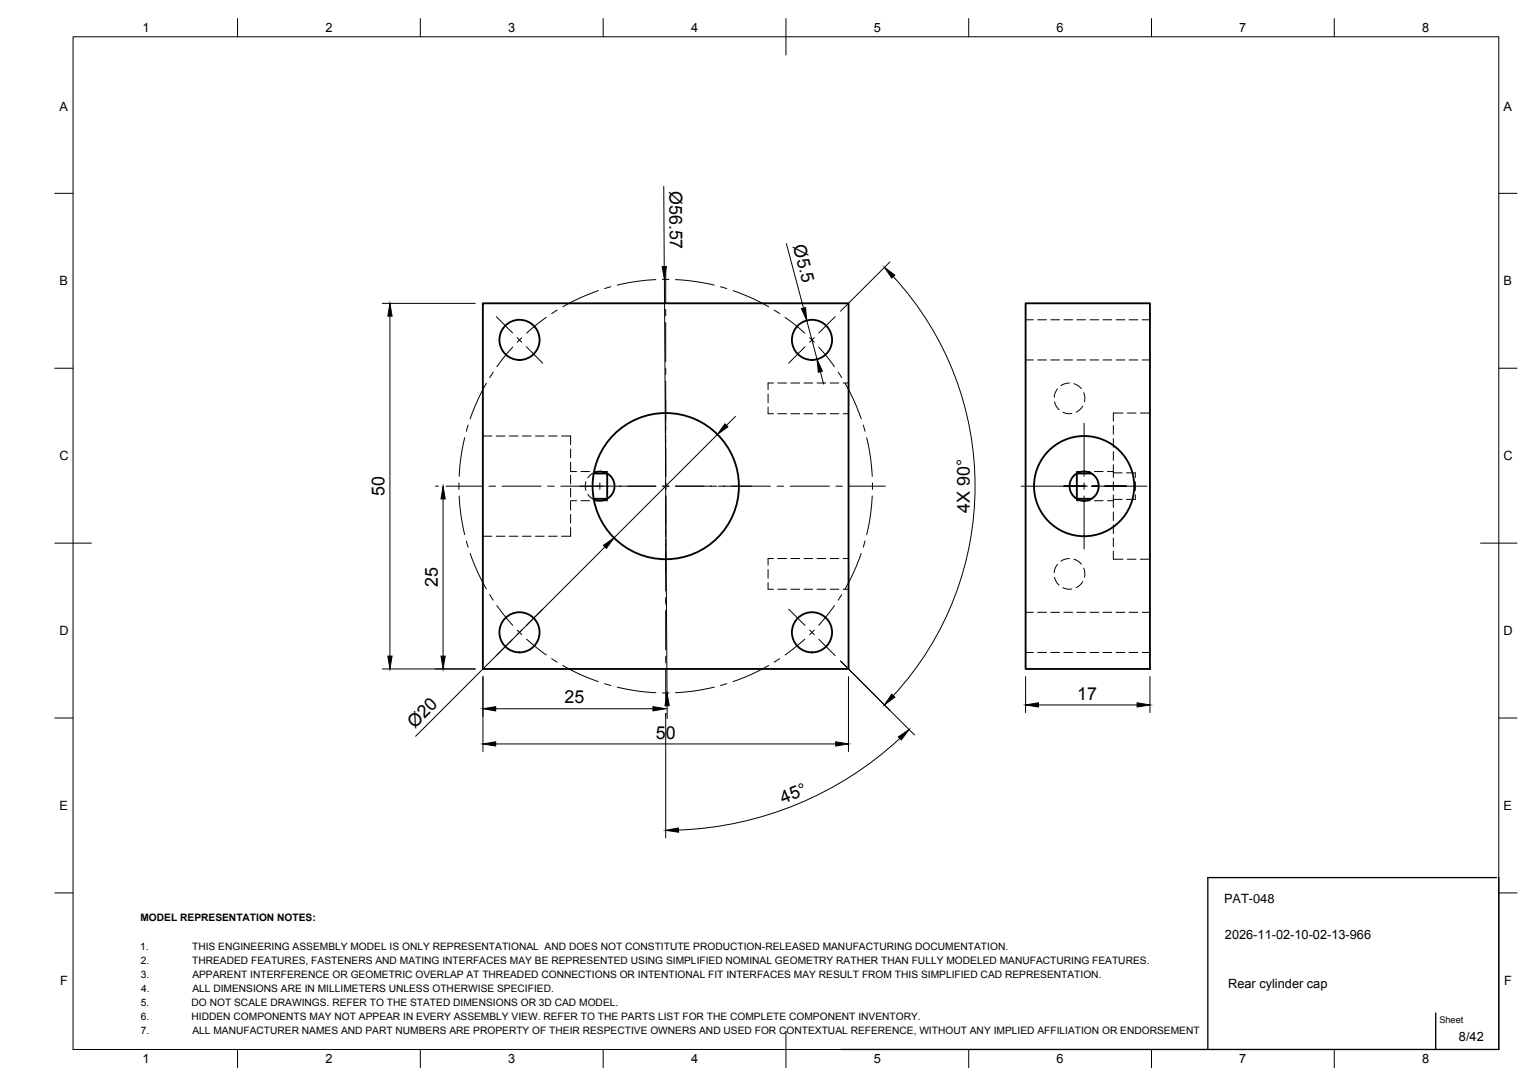
ISO-10303-21;
HEADER;
/* Generated by software containing ST-Developer
 * from STEP Tools, Inc. (www.steptools.com) 
 */

FILE_DESCRIPTION(
/* description */ ('Guided pneumatic stop gate'),
/* implementation_level */ '2;1');

FILE_NAME(
/* name */ 'Rear cylinder cap.step',
/* time_stamp */ '2026-10-27T21:43:45-07:00',
/* author */ (''),
/* organization */ (''),
/* preprocessor_version */ 'ST-DEVELOPER v20.2',
/* originating_system */ 'Autodesk Translation Framework v15.17.0.0',
/* authorisation */ '');

FILE_SCHEMA (('AUTOMOTIVE_DESIGN { 1 0 10303 214 3 1 1 }'));
ENDSEC;

DATA;
#10=MECHANICAL_DESIGN_GEOMETRIC_PRESENTATION_REPRESENTATION('',(#538),#14392);
#454=SHAPE_REPRESENTATION_RELATIONSHIP('SRR','None',#14588,#496);
#496=ADVANCED_BREP_SHAPE_REPRESENTATION('',(#580),#14350);
#538=STYLED_ITEM('',(#14877),#580);
#580=MANIFOLD_SOLID_BREP('Body1',#7878);
#640=FACE_BOUND('',#1705,.T.);
#641=FACE_BOUND('',#1712,.T.);
#642=FACE_BOUND('',#1713,.T.);
#643=FACE_BOUND('',#1714,.T.);
#644=FACE_BOUND('',#1715,.T.);
#645=FACE_BOUND('',#1718,.T.);
#646=FACE_BOUND('',#1719,.T.);
#647=FACE_BOUND('',#1720,.T.);
#648=FACE_BOUND('',#1721,.T.);
#649=FACE_BOUND('',#1722,.T.);
#650=FACE_BOUND('',#1725,.T.);
#651=FACE_BOUND('',#1727,.T.);
#652=FACE_BOUND('',#1728,.T.);
#832=ELLIPSE('',#8530,0.282842712474618,0.2);
#833=ELLIPSE('',#8531,0.282842712474618,0.2);
#834=ELLIPSE('',#8532,0.282842712474618,0.2);
#835=ELLIPSE('',#8535,0.282842712474618,0.2);
#836=ELLIPSE('',#8536,0.282842712474618,0.2);
#837=ELLIPSE('',#8538,0.282842712474618,0.2);
#838=ELLIPSE('',#8539,0.282842712474618,0.2);
#880=PLANE('',#8516);
#881=PLANE('',#8520);
#882=PLANE('',#8521);
#883=PLANE('',#8523);
#884=PLANE('',#8525);
#885=PLANE('',#8540);
#886=PLANE('',#8542);
#887=PLANE('',#8544);
#888=PLANE('',#8546);
#889=PLANE('',#8552);
#890=PLANE('',#8558);
#891=PLANE('',#8573);
#892=PLANE('',#8574);
#893=PLANE('',#8575);
#894=PLANE('',#8576);
#895=PLANE('',#8577);
#896=PLANE('',#8578);
#1185=FACE_OUTER_BOUND('',#1685,.T.);
#1186=FACE_OUTER_BOUND('',#1686,.T.);
#1187=FACE_OUTER_BOUND('',#1687,.T.);
#1188=FACE_OUTER_BOUND('',#1688,.T.);
#1189=FACE_OUTER_BOUND('',#1689,.T.);
#1190=FACE_OUTER_BOUND('',#1690,.T.);
#1191=FACE_OUTER_BOUND('',#1691,.T.);
#1192=FACE_OUTER_BOUND('',#1692,.T.);
#1193=FACE_OUTER_BOUND('',#1693,.T.);
#1194=FACE_OUTER_BOUND('',#1694,.T.);
#1195=FACE_OUTER_BOUND('',#1695,.T.);
#1196=FACE_OUTER_BOUND('',#1696,.T.);
#1197=FACE_OUTER_BOUND('',#1697,.T.);
#1198=FACE_OUTER_BOUND('',#1698,.T.);
#1199=FACE_OUTER_BOUND('',#1699,.T.);
#1200=FACE_OUTER_BOUND('',#1700,.T.);
#1201=FACE_OUTER_BOUND('',#1701,.T.);
#1202=FACE_OUTER_BOUND('',#1702,.T.);
#1203=FACE_OUTER_BOUND('',#1703,.T.);
#1204=FACE_OUTER_BOUND('',#1704,.T.);
#1205=FACE_OUTER_BOUND('',#1706,.T.);
#1206=FACE_OUTER_BOUND('',#1707,.T.);
#1207=FACE_OUTER_BOUND('',#1708,.T.);
#1208=FACE_OUTER_BOUND('',#1709,.T.);
#1209=FACE_OUTER_BOUND('',#1710,.T.);
#1210=FACE_OUTER_BOUND('',#1711,.T.);
#1211=FACE_OUTER_BOUND('',#1716,.T.);
#1212=FACE_OUTER_BOUND('',#1717,.T.);
#1213=FACE_OUTER_BOUND('',#1723,.T.);
#1214=FACE_OUTER_BOUND('',#1724,.T.);
#1215=FACE_OUTER_BOUND('',#1726,.T.);
#1685=EDGE_LOOP('',(#5592,#5593,#5594,#5595));
#1686=EDGE_LOOP('',(#5596));
#1687=EDGE_LOOP('',(#5597,#5598,#5599,#5600));
#1688=EDGE_LOOP('',(#5601));
#1689=EDGE_LOOP('',(#5602,#5603));
#1690=EDGE_LOOP('',(#5604,#5605));
#1691=EDGE_LOOP('',(#5606,#5607));
#1692=EDGE_LOOP('',(#5608,#5609,#5610,#5611,#5612,#5613,#5614,#5615,#5616,
#5617,#5618,#5619,#5620));
#1693=EDGE_LOOP('',(#5621,#5622,#5623));
#1694=EDGE_LOOP('',(#5624,#5625,#5626));
#1695=EDGE_LOOP('',(#5627,#5628));
#1696=EDGE_LOOP('',(#5629,#5630));
#1697=EDGE_LOOP('',(#5631,#5632));
#1698=EDGE_LOOP('',(#5633,#5634));
#1699=EDGE_LOOP('',(#5635,#5636,#5637));
#1700=EDGE_LOOP('',(#5638,#5639,#5640));
#1701=EDGE_LOOP('',(#5641,#5642,#5643,#5644,#5645,#5646,#5647,#5648,#5649));
#1702=EDGE_LOOP('',(#5650,#5651,#5652,#5653));
#1703=EDGE_LOOP('',(#5654,#5655,#5656,#5657));
#1704=EDGE_LOOP('',(#5658));
#1705=EDGE_LOOP('',(#5659));
#1706=EDGE_LOOP('',(#5660,#5661,#5662,#5663));
#1707=EDGE_LOOP('',(#5664,#5665,#5666,#5667));
#1708=EDGE_LOOP('',(#5668,#5669,#5670,#5671));
#1709=EDGE_LOOP('',(#5672,#5673,#5674,#5675));
#1710=EDGE_LOOP('',(#5676,#5677,#5678,#5679,#5680,#5681,#5682,#5683));
#1711=EDGE_LOOP('',(#5684,#5685,#5686,#5687));
#1712=EDGE_LOOP('',(#5688));
#1713=EDGE_LOOP('',(#5689));
#1714=EDGE_LOOP('',(#5690));
#1715=EDGE_LOOP('',(#5691));
#1716=EDGE_LOOP('',(#5692,#5693,#5694,#5695));
#1717=EDGE_LOOP('',(#5696,#5697,#5698,#5699));
#1718=EDGE_LOOP('',(#5700));
#1719=EDGE_LOOP('',(#5701));
#1720=EDGE_LOOP('',(#5702));
#1721=EDGE_LOOP('',(#5703));
#1722=EDGE_LOOP('',(#5704));
#1723=EDGE_LOOP('',(#5705,#5706,#5707,#5708));
#1724=EDGE_LOOP('',(#5709,#5710,#5711,#5712));
#1725=EDGE_LOOP('',(#5713));
#1726=EDGE_LOOP('',(#5714,#5715,#5716,#5717));
#1727=EDGE_LOOP('',(#5718));
#1728=EDGE_LOOP('',(#5719));
#2360=LINE('',#12221,#2905);
#2361=LINE('',#12228,#2906);
#2362=LINE('',#12234,#2907);
#2363=LINE('',#12238,#2908);
#2364=LINE('',#12242,#2909);
#2365=LINE('',#12247,#2910);
#2366=LINE('',#12251,#2911);
#2367=LINE('',#12255,#2912);
#2368=LINE('',#12260,#2913);
#2369=LINE('',#12262,#2914);
#2370=LINE('',#12283,#2915);
#2371=LINE('',#12293,#2916);
#2372=LINE('',#12300,#2917);
#2373=LINE('',#12306,#2918);
#2374=LINE('',#12312,#2919);
#2375=LINE('',#12318,#2920);
#2376=LINE('',#12323,#2921);
#2377=LINE('',#12327,#2922);
#2378=LINE('',#12329,#2923);
#2379=LINE('',#12331,#2924);
#2380=LINE('',#12332,#2925);
#2381=LINE('',#12335,#2926);
#2382=LINE('',#12337,#2927);
#2383=LINE('',#12338,#2928);
#2384=LINE('',#12341,#2929);
#2385=LINE('',#12343,#2930);
#2386=LINE('',#12344,#2931);
#2387=LINE('',#12346,#2932);
#2388=LINE('',#12347,#2933);
#2905=VECTOR('',#9725,0.21);
#2906=VECTOR('',#9734,0.21);
#2907=VECTOR('',#9741,1.);
#2908=VECTOR('',#9746,1.);
#2909=VECTOR('',#9751,1.);
#2910=VECTOR('',#9756,1.);
#2911=VECTOR('',#9759,1.);
#2912=VECTOR('',#9762,0.2);
#2913=VECTOR('',#9767,1.);
#2914=VECTOR('',#9768,1.);
#2915=VECTOR('',#9807,0.2);
#2916=VECTOR('',#9820,0.685);
#2917=VECTOR('',#9829,0.275);
#2918=VECTOR('',#9836,0.275);
#2919=VECTOR('',#9843,0.275);
#2920=VECTOR('',#9850,0.275);
#2921=VECTOR('',#9857,1.);
#2922=VECTOR('',#9860,1.);
#2923=VECTOR('',#9861,1.);
#2924=VECTOR('',#9862,1.);
#2925=VECTOR('',#9863,1.);
#2926=VECTOR('',#9866,1.);
#2927=VECTOR('',#9867,1.);
#2928=VECTOR('',#9868,1.);
#2929=VECTOR('',#9871,1.);
#2930=VECTOR('',#9872,1.);
#2931=VECTOR('',#9873,1.);
#2932=VECTOR('',#9876,1.);
#2933=VECTOR('',#9877,1.);
#3417=CIRCLE('',#8514,0.21);
#3418=CIRCLE('',#8515,0.21);
#3419=CIRCLE('',#8518,0.21);
#3420=CIRCLE('',#8519,0.21);
#3421=CIRCLE('',#8522,0.2);
#3422=CIRCLE('',#8524,0.2);
#3423=CIRCLE('',#8526,0.2);
#3424=CIRCLE('',#8528,0.2);
#3425=CIRCLE('',#8529,0.2);
#3426=CIRCLE('',#8533,0.2);
#3427=CIRCLE('',#8541,1.);
#3428=CIRCLE('',#8543,0.2);
#3429=CIRCLE('',#8545,0.2);
#3430=CIRCLE('',#8547,0.2);
#3431=CIRCLE('',#8551,0.2);
#3432=CIRCLE('',#8553,1.);
#3433=CIRCLE('',#8554,1.);
#3434=CIRCLE('',#8556,0.685);
#3435=CIRCLE('',#8557,0.685);
#3436=CIRCLE('',#8560,0.275);
#3437=CIRCLE('',#8561,0.275);
#3438=CIRCLE('',#8563,0.275);
#3439=CIRCLE('',#8564,0.275);
#3440=CIRCLE('',#8566,0.275);
#3441=CIRCLE('',#8567,0.275);
#3442=CIRCLE('',#8569,0.275);
#3443=CIRCLE('',#8570,0.275);
#3444=CIRCLE('',#8572,1.);
#3823=VERTEX_POINT('',#12218);
#3824=VERTEX_POINT('',#12220);
#3825=VERTEX_POINT('',#12225);
#3826=VERTEX_POINT('',#12227);
#3827=VERTEX_POINT('',#12232);
#3828=VERTEX_POINT('',#12233);
#3829=VERTEX_POINT('',#12237);
#3830=VERTEX_POINT('',#12241);
#3831=VERTEX_POINT('',#12245);
#3832=VERTEX_POINT('',#12246);
#3833=VERTEX_POINT('',#12248);
#3834=VERTEX_POINT('',#12250);
#3835=VERTEX_POINT('',#12252);
#3836=VERTEX_POINT('',#12254);
#3837=VERTEX_POINT('',#12256);
#3838=VERTEX_POINT('',#12258);
#3839=VERTEX_POINT('',#12261);
#3840=VERTEX_POINT('',#12282);
#3841=VERTEX_POINT('',#12286);
#3842=VERTEX_POINT('',#12290);
#3843=VERTEX_POINT('',#12292);
#3844=VERTEX_POINT('',#12297);
#3845=VERTEX_POINT('',#12299);
#3846=VERTEX_POINT('',#12303);
#3847=VERTEX_POINT('',#12305);
#3848=VERTEX_POINT('',#12309);
#3849=VERTEX_POINT('',#12311);
#3850=VERTEX_POINT('',#12315);
#3851=VERTEX_POINT('',#12317);
#3852=VERTEX_POINT('',#12321);
#3853=VERTEX_POINT('',#12325);
#3854=VERTEX_POINT('',#12326);
#3855=VERTEX_POINT('',#12328);
#3856=VERTEX_POINT('',#12330);
#3857=VERTEX_POINT('',#12334);
#3858=VERTEX_POINT('',#12336);
#3859=VERTEX_POINT('',#12340);
#3860=VERTEX_POINT('',#12342);
#4494=EDGE_CURVE('',#3823,#3823,#3417,.T.);
#4495=EDGE_CURVE('',#3823,#3824,#2360,.T.);
#4496=EDGE_CURVE('',#3824,#3824,#3418,.T.);
#4497=EDGE_CURVE('',#3825,#3825,#3419,.T.);
#4498=EDGE_CURVE('',#3825,#3826,#2361,.T.);
#4499=EDGE_CURVE('',#3826,#3826,#3420,.T.);
#4500=EDGE_CURVE('',#3827,#3828,#2362,.T.);
#4501=EDGE_CURVE('',#3828,#3827,#3421,.T.);
#4502=EDGE_CURVE('',#3828,#3829,#2363,.T.);
#4503=EDGE_CURVE('',#3829,#3828,#3422,.T.);
#4504=EDGE_CURVE('',#3830,#3827,#2364,.T.);
#4505=EDGE_CURVE('',#3827,#3830,#3423,.T.);
#4506=EDGE_CURVE('',#3831,#3832,#2365,.T.);
#4507=EDGE_CURVE('',#3833,#3831,#3424,.T.);
#4508=EDGE_CURVE('',#3834,#3833,#2366,.T.);
#4509=EDGE_CURVE('',#3835,#3834,#3425,.T.);
#4510=EDGE_CURVE('',#3835,#3836,#2367,.T.);
#4511=EDGE_CURVE('',#3837,#3836,#832,.T.);
#4512=EDGE_CURVE('',#3838,#3837,#833,.T.);
#4513=EDGE_CURVE('',#3828,#3838,#2368,.T.);
#4514=EDGE_CURVE('',#3839,#3827,#2369,.T.);
#4515=EDGE_CURVE('',#3836,#3839,#834,.T.);
#4516=EDGE_CURVE('',#3832,#3835,#3426,.T.);
#4517=EDGE_CURVE('',#3829,#3837,#835,.T.);
#4518=EDGE_CURVE('',#3837,#3828,#836,.T.);
#4519=EDGE_CURVE('',#3836,#3830,#837,.T.);
#4520=EDGE_CURVE('',#3827,#3836,#838,.T.);
#4521=EDGE_CURVE('',#3833,#3831,#3427,.T.);
#4522=EDGE_CURVE('',#3828,#3827,#3428,.T.);
#4523=EDGE_CURVE('',#3838,#3828,#3429,.T.);
#4524=EDGE_CURVE('',#3827,#3839,#3430,.T.);
#4525=EDGE_CURVE('',#3836,#3840,#2370,.T.);
#4526=EDGE_CURVE('',#3840,#3840,#3431,.T.);
#4527=EDGE_CURVE('',#3841,#3834,#3432,.T.);
#4528=EDGE_CURVE('',#3832,#3841,#3433,.T.);
#4529=EDGE_CURVE('',#3842,#3842,#3434,.T.);
#4530=EDGE_CURVE('',#3842,#3843,#2371,.T.);
#4531=EDGE_CURVE('',#3843,#3843,#3435,.T.);
#4532=EDGE_CURVE('',#3844,#3844,#3436,.T.);
#4533=EDGE_CURVE('',#3844,#3845,#2372,.T.);
#4534=EDGE_CURVE('',#3845,#3845,#3437,.T.);
#4535=EDGE_CURVE('',#3846,#3846,#3438,.T.);
#4536=EDGE_CURVE('',#3846,#3847,#2373,.T.);
#4537=EDGE_CURVE('',#3847,#3847,#3439,.T.);
#4538=EDGE_CURVE('',#3848,#3848,#3440,.T.);
#4539=EDGE_CURVE('',#3848,#3849,#2374,.T.);
#4540=EDGE_CURVE('',#3849,#3849,#3441,.T.);
#4541=EDGE_CURVE('',#3850,#3850,#3442,.T.);
#4542=EDGE_CURVE('',#3850,#3851,#2375,.T.);
#4543=EDGE_CURVE('',#3851,#3851,#3443,.T.);
#4544=EDGE_CURVE('',#3852,#3852,#3444,.T.);
#4545=EDGE_CURVE('',#3852,#3841,#2376,.T.);
#4546=EDGE_CURVE('',#3853,#3854,#2377,.T.);
#4547=EDGE_CURVE('',#3854,#3855,#2378,.T.);
#4548=EDGE_CURVE('',#3856,#3855,#2379,.T.);
#4549=EDGE_CURVE('',#3853,#3856,#2380,.T.);
#4550=EDGE_CURVE('',#3857,#3853,#2381,.T.);
#4551=EDGE_CURVE('',#3858,#3856,#2382,.T.);
#4552=EDGE_CURVE('',#3857,#3858,#2383,.T.);
#4553=EDGE_CURVE('',#3859,#3857,#2384,.T.);
#4554=EDGE_CURVE('',#3860,#3858,#2385,.T.);
#4555=EDGE_CURVE('',#3859,#3860,#2386,.T.);
#4556=EDGE_CURVE('',#3854,#3859,#2387,.T.);
#4557=EDGE_CURVE('',#3855,#3860,#2388,.T.);
#5592=ORIENTED_EDGE('',*,*,#4494,.F.);
#5593=ORIENTED_EDGE('',*,*,#4495,.T.);
#5594=ORIENTED_EDGE('',*,*,#4496,.T.);
#5595=ORIENTED_EDGE('',*,*,#4495,.F.);
#5596=ORIENTED_EDGE('',*,*,#4496,.F.);
#5597=ORIENTED_EDGE('',*,*,#4497,.F.);
#5598=ORIENTED_EDGE('',*,*,#4498,.T.);
#5599=ORIENTED_EDGE('',*,*,#4499,.T.);
#5600=ORIENTED_EDGE('',*,*,#4498,.F.);
#5601=ORIENTED_EDGE('',*,*,#4499,.F.);
#5602=ORIENTED_EDGE('',*,*,#4500,.F.);
#5603=ORIENTED_EDGE('',*,*,#4501,.F.);
#5604=ORIENTED_EDGE('',*,*,#4502,.F.);
#5605=ORIENTED_EDGE('',*,*,#4503,.F.);
#5606=ORIENTED_EDGE('',*,*,#4504,.F.);
#5607=ORIENTED_EDGE('',*,*,#4505,.F.);
#5608=ORIENTED_EDGE('',*,*,#4506,.F.);
#5609=ORIENTED_EDGE('',*,*,#4507,.F.);
#5610=ORIENTED_EDGE('',*,*,#4508,.F.);
#5611=ORIENTED_EDGE('',*,*,#4509,.F.);
#5612=ORIENTED_EDGE('',*,*,#4510,.T.);
#5613=ORIENTED_EDGE('',*,*,#4511,.F.);
#5614=ORIENTED_EDGE('',*,*,#4512,.F.);
#5615=ORIENTED_EDGE('',*,*,#4513,.F.);
#5616=ORIENTED_EDGE('',*,*,#4501,.T.);
#5617=ORIENTED_EDGE('',*,*,#4514,.F.);
#5618=ORIENTED_EDGE('',*,*,#4515,.F.);
#5619=ORIENTED_EDGE('',*,*,#4510,.F.);
#5620=ORIENTED_EDGE('',*,*,#4516,.F.);
#5621=ORIENTED_EDGE('',*,*,#4517,.F.);
#5622=ORIENTED_EDGE('',*,*,#4503,.T.);
#5623=ORIENTED_EDGE('',*,*,#4518,.F.);
#5624=ORIENTED_EDGE('',*,*,#4519,.F.);
#5625=ORIENTED_EDGE('',*,*,#4520,.F.);
#5626=ORIENTED_EDGE('',*,*,#4505,.T.);
#5627=ORIENTED_EDGE('',*,*,#4521,.F.);
#5628=ORIENTED_EDGE('',*,*,#4507,.T.);
#5629=ORIENTED_EDGE('',*,*,#4500,.T.);
#5630=ORIENTED_EDGE('',*,*,#4522,.T.);
#5631=ORIENTED_EDGE('',*,*,#4513,.T.);
#5632=ORIENTED_EDGE('',*,*,#4523,.T.);
#5633=ORIENTED_EDGE('',*,*,#4514,.T.);
#5634=ORIENTED_EDGE('',*,*,#4524,.T.);
#5635=ORIENTED_EDGE('',*,*,#4518,.T.);
#5636=ORIENTED_EDGE('',*,*,#4523,.F.);
#5637=ORIENTED_EDGE('',*,*,#4512,.T.);
#5638=ORIENTED_EDGE('',*,*,#4515,.T.);
#5639=ORIENTED_EDGE('',*,*,#4524,.F.);
#5640=ORIENTED_EDGE('',*,*,#4520,.T.);
#5641=ORIENTED_EDGE('',*,*,#4504,.T.);
#5642=ORIENTED_EDGE('',*,*,#4522,.F.);
#5643=ORIENTED_EDGE('',*,*,#4502,.T.);
#5644=ORIENTED_EDGE('',*,*,#4517,.T.);
#5645=ORIENTED_EDGE('',*,*,#4511,.T.);
#5646=ORIENTED_EDGE('',*,*,#4525,.T.);
#5647=ORIENTED_EDGE('',*,*,#4526,.F.);
#5648=ORIENTED_EDGE('',*,*,#4525,.F.);
#5649=ORIENTED_EDGE('',*,*,#4519,.T.);
#5650=ORIENTED_EDGE('',*,*,#4516,.T.);
#5651=ORIENTED_EDGE('',*,*,#4509,.T.);
#5652=ORIENTED_EDGE('',*,*,#4527,.F.);
#5653=ORIENTED_EDGE('',*,*,#4528,.F.);
#5654=ORIENTED_EDGE('',*,*,#4529,.F.);
#5655=ORIENTED_EDGE('',*,*,#4530,.T.);
#5656=ORIENTED_EDGE('',*,*,#4531,.F.);
#5657=ORIENTED_EDGE('',*,*,#4530,.F.);
#5658=ORIENTED_EDGE('',*,*,#4529,.T.);
#5659=ORIENTED_EDGE('',*,*,#4526,.T.);
#5660=ORIENTED_EDGE('',*,*,#4532,.F.);
#5661=ORIENTED_EDGE('',*,*,#4533,.T.);
#5662=ORIENTED_EDGE('',*,*,#4534,.F.);
#5663=ORIENTED_EDGE('',*,*,#4533,.F.);
#5664=ORIENTED_EDGE('',*,*,#4535,.F.);
#5665=ORIENTED_EDGE('',*,*,#4536,.T.);
#5666=ORIENTED_EDGE('',*,*,#4537,.F.);
#5667=ORIENTED_EDGE('',*,*,#4536,.F.);
#5668=ORIENTED_EDGE('',*,*,#4538,.F.);
#5669=ORIENTED_EDGE('',*,*,#4539,.T.);
#5670=ORIENTED_EDGE('',*,*,#4540,.F.);
#5671=ORIENTED_EDGE('',*,*,#4539,.F.);
#5672=ORIENTED_EDGE('',*,*,#4541,.F.);
#5673=ORIENTED_EDGE('',*,*,#4542,.T.);
#5674=ORIENTED_EDGE('',*,*,#4543,.F.);
#5675=ORIENTED_EDGE('',*,*,#4542,.F.);
#5676=ORIENTED_EDGE('',*,*,#4544,.F.);
#5677=ORIENTED_EDGE('',*,*,#4545,.T.);
#5678=ORIENTED_EDGE('',*,*,#4527,.T.);
#5679=ORIENTED_EDGE('',*,*,#4508,.T.);
#5680=ORIENTED_EDGE('',*,*,#4521,.T.);
#5681=ORIENTED_EDGE('',*,*,#4506,.T.);
#5682=ORIENTED_EDGE('',*,*,#4528,.T.);
#5683=ORIENTED_EDGE('',*,*,#4545,.F.);
#5684=ORIENTED_EDGE('',*,*,#4546,.T.);
#5685=ORIENTED_EDGE('',*,*,#4547,.T.);
#5686=ORIENTED_EDGE('',*,*,#4548,.F.);
#5687=ORIENTED_EDGE('',*,*,#4549,.F.);
#5688=ORIENTED_EDGE('',*,*,#4534,.T.);
#5689=ORIENTED_EDGE('',*,*,#4537,.T.);
#5690=ORIENTED_EDGE('',*,*,#4540,.T.);
#5691=ORIENTED_EDGE('',*,*,#4543,.T.);
#5692=ORIENTED_EDGE('',*,*,#4550,.T.);
#5693=ORIENTED_EDGE('',*,*,#4549,.T.);
#5694=ORIENTED_EDGE('',*,*,#4551,.F.);
#5695=ORIENTED_EDGE('',*,*,#4552,.F.);
#5696=ORIENTED_EDGE('',*,*,#4553,.T.);
#5697=ORIENTED_EDGE('',*,*,#4552,.T.);
#5698=ORIENTED_EDGE('',*,*,#4554,.F.);
#5699=ORIENTED_EDGE('',*,*,#4555,.F.);
#5700=ORIENTED_EDGE('',*,*,#4544,.T.);
#5701=ORIENTED_EDGE('',*,*,#4541,.T.);
#5702=ORIENTED_EDGE('',*,*,#4538,.T.);
#5703=ORIENTED_EDGE('',*,*,#4535,.T.);
#5704=ORIENTED_EDGE('',*,*,#4532,.T.);
#5705=ORIENTED_EDGE('',*,*,#4556,.T.);
#5706=ORIENTED_EDGE('',*,*,#4555,.T.);
#5707=ORIENTED_EDGE('',*,*,#4557,.F.);
#5708=ORIENTED_EDGE('',*,*,#4547,.F.);
#5709=ORIENTED_EDGE('',*,*,#4557,.T.);
#5710=ORIENTED_EDGE('',*,*,#4554,.T.);
#5711=ORIENTED_EDGE('',*,*,#4551,.T.);
#5712=ORIENTED_EDGE('',*,*,#4548,.T.);
#5713=ORIENTED_EDGE('',*,*,#4531,.T.);
#5714=ORIENTED_EDGE('',*,*,#4556,.F.);
#5715=ORIENTED_EDGE('',*,*,#4546,.F.);
#5716=ORIENTED_EDGE('',*,*,#4550,.F.);
#5717=ORIENTED_EDGE('',*,*,#4553,.F.);
#5718=ORIENTED_EDGE('',*,*,#4494,.T.);
#5719=ORIENTED_EDGE('',*,*,#4497,.T.);
#7260=CYLINDRICAL_SURFACE('',#8513,0.21);
#7261=CYLINDRICAL_SURFACE('',#8517,0.21);
#7262=CYLINDRICAL_SURFACE('',#8527,0.2);
#7263=CYLINDRICAL_SURFACE('',#8534,0.2);
#7264=CYLINDRICAL_SURFACE('',#8537,0.2);
#7265=CYLINDRICAL_SURFACE('',#8548,0.2);
#7266=CYLINDRICAL_SURFACE('',#8549,0.2);
#7267=CYLINDRICAL_SURFACE('',#8550,0.2);
#7268=CYLINDRICAL_SURFACE('',#8555,0.685);
#7269=CYLINDRICAL_SURFACE('',#8559,0.275);
#7270=CYLINDRICAL_SURFACE('',#8562,0.275);
#7271=CYLINDRICAL_SURFACE('',#8565,0.275);
#7272=CYLINDRICAL_SURFACE('',#8568,0.275);
#7273=CYLINDRICAL_SURFACE('',#8571,1.);
#7467=ADVANCED_FACE('',(#1185),#7260,.F.);
#7468=ADVANCED_FACE('',(#1186),#880,.F.);
#7469=ADVANCED_FACE('',(#1187),#7261,.F.);
#7470=ADVANCED_FACE('',(#1188),#881,.F.);
#7471=ADVANCED_FACE('',(#1189),#882,.F.);
#7472=ADVANCED_FACE('',(#1190),#883,.F.);
#7473=ADVANCED_FACE('',(#1191),#884,.F.);
#7474=ADVANCED_FACE('',(#1192),#7262,.F.);
#7475=ADVANCED_FACE('',(#1193),#7263,.F.);
#7476=ADVANCED_FACE('',(#1194),#7264,.F.);
#7477=ADVANCED_FACE('',(#1195),#885,.T.);
#7478=ADVANCED_FACE('',(#1196),#886,.T.);
#7479=ADVANCED_FACE('',(#1197),#887,.T.);
#7480=ADVANCED_FACE('',(#1198),#888,.T.);
#7481=ADVANCED_FACE('',(#1199),#7265,.F.);
#7482=ADVANCED_FACE('',(#1200),#7266,.F.);
#7483=ADVANCED_FACE('',(#1201),#7267,.F.);
#7484=ADVANCED_FACE('',(#1202),#889,.F.);
#7485=ADVANCED_FACE('',(#1203),#7268,.F.);
#7486=ADVANCED_FACE('',(#1204,#640),#890,.T.);
#7487=ADVANCED_FACE('',(#1205),#7269,.F.);
#7488=ADVANCED_FACE('',(#1206),#7270,.F.);
#7489=ADVANCED_FACE('',(#1207),#7271,.F.);
#7490=ADVANCED_FACE('',(#1208),#7272,.F.);
#7491=ADVANCED_FACE('',(#1209),#7273,.F.);
#7492=ADVANCED_FACE('',(#1210,#641,#642,#643,#644),#891,.T.);
#7493=ADVANCED_FACE('',(#1211),#892,.T.);
#7494=ADVANCED_FACE('',(#1212,#645,#646,#647,#648,#649),#893,.T.);
#7495=ADVANCED_FACE('',(#1213),#894,.T.);
#7496=ADVANCED_FACE('',(#1214,#650),#895,.T.);
#7497=ADVANCED_FACE('',(#1215,#651,#652),#896,.F.);
#7878=CLOSED_SHELL('',(#7467,#7468,#7469,#7470,#7471,#7472,#7473,#7474,
#7475,#7476,#7477,#7478,#7479,#7480,#7481,#7482,#7483,#7484,#7485,#7486,
#7487,#7488,#7489,#7490,#7491,#7492,#7493,#7494,#7495,#7496,#7497));
#8512=AXIS2_PLACEMENT_3D('',#12216,#9719,#9720);
#8513=AXIS2_PLACEMENT_3D('',#12217,#9721,#9722);
#8514=AXIS2_PLACEMENT_3D('',#12219,#9723,#9724);
#8515=AXIS2_PLACEMENT_3D('',#12222,#9726,#9727);
#8516=AXIS2_PLACEMENT_3D('',#12223,#9728,#9729);
#8517=AXIS2_PLACEMENT_3D('',#12224,#9730,#9731);
#8518=AXIS2_PLACEMENT_3D('',#12226,#9732,#9733);
#8519=AXIS2_PLACEMENT_3D('',#12229,#9735,#9736);
#8520=AXIS2_PLACEMENT_3D('',#12230,#9737,#9738);
#8521=AXIS2_PLACEMENT_3D('',#12231,#9739,#9740);
#8522=AXIS2_PLACEMENT_3D('',#12235,#9742,#9743);
#8523=AXIS2_PLACEMENT_3D('',#12236,#9744,#9745);
#8524=AXIS2_PLACEMENT_3D('',#12239,#9747,#9748);
#8525=AXIS2_PLACEMENT_3D('',#12240,#9749,#9750);
#8526=AXIS2_PLACEMENT_3D('',#12243,#9752,#9753);
#8527=AXIS2_PLACEMENT_3D('',#12244,#9754,#9755);
#8528=AXIS2_PLACEMENT_3D('',#12249,#9757,#9758);
#8529=AXIS2_PLACEMENT_3D('',#12253,#9760,#9761);
#8530=AXIS2_PLACEMENT_3D('',#12257,#9763,#9764);
#8531=AXIS2_PLACEMENT_3D('',#12259,#9765,#9766);
#8532=AXIS2_PLACEMENT_3D('',#12263,#9769,#9770);
#8533=AXIS2_PLACEMENT_3D('',#12264,#9771,#9772);
#8534=AXIS2_PLACEMENT_3D('',#12265,#9773,#9774);
#8535=AXIS2_PLACEMENT_3D('',#12266,#9775,#9776);
#8536=AXIS2_PLACEMENT_3D('',#12267,#9777,#9778);
#8537=AXIS2_PLACEMENT_3D('',#12268,#9779,#9780);
#8538=AXIS2_PLACEMENT_3D('',#12269,#9781,#9782);
#8539=AXIS2_PLACEMENT_3D('',#12270,#9783,#9784);
#8540=AXIS2_PLACEMENT_3D('',#12271,#9785,#9786);
#8541=AXIS2_PLACEMENT_3D('',#12272,#9787,#9788);
#8542=AXIS2_PLACEMENT_3D('',#12273,#9789,#9790);
#8543=AXIS2_PLACEMENT_3D('',#12274,#9791,#9792);
#8544=AXIS2_PLACEMENT_3D('',#12275,#9793,#9794);
#8545=AXIS2_PLACEMENT_3D('',#12276,#9795,#9796);
#8546=AXIS2_PLACEMENT_3D('',#12277,#9797,#9798);
#8547=AXIS2_PLACEMENT_3D('',#12278,#9799,#9800);
#8548=AXIS2_PLACEMENT_3D('',#12279,#9801,#9802);
#8549=AXIS2_PLACEMENT_3D('',#12280,#9803,#9804);
#8550=AXIS2_PLACEMENT_3D('',#12281,#9805,#9806);
#8551=AXIS2_PLACEMENT_3D('',#12284,#9808,#9809);
#8552=AXIS2_PLACEMENT_3D('',#12285,#9810,#9811);
#8553=AXIS2_PLACEMENT_3D('',#12287,#9812,#9813);
#8554=AXIS2_PLACEMENT_3D('',#12288,#9814,#9815);
#8555=AXIS2_PLACEMENT_3D('',#12289,#9816,#9817);
#8556=AXIS2_PLACEMENT_3D('',#12291,#9818,#9819);
#8557=AXIS2_PLACEMENT_3D('',#12294,#9821,#9822);
#8558=AXIS2_PLACEMENT_3D('',#12295,#9823,#9824);
#8559=AXIS2_PLACEMENT_3D('',#12296,#9825,#9826);
#8560=AXIS2_PLACEMENT_3D('',#12298,#9827,#9828);
#8561=AXIS2_PLACEMENT_3D('',#12301,#9830,#9831);
#8562=AXIS2_PLACEMENT_3D('',#12302,#9832,#9833);
#8563=AXIS2_PLACEMENT_3D('',#12304,#9834,#9835);
#8564=AXIS2_PLACEMENT_3D('',#12307,#9837,#9838);
#8565=AXIS2_PLACEMENT_3D('',#12308,#9839,#9840);
#8566=AXIS2_PLACEMENT_3D('',#12310,#9841,#9842);
#8567=AXIS2_PLACEMENT_3D('',#12313,#9844,#9845);
#8568=AXIS2_PLACEMENT_3D('',#12314,#9846,#9847);
#8569=AXIS2_PLACEMENT_3D('',#12316,#9848,#9849);
#8570=AXIS2_PLACEMENT_3D('',#12319,#9851,#9852);
#8571=AXIS2_PLACEMENT_3D('',#12320,#9853,#9854);
#8572=AXIS2_PLACEMENT_3D('',#12322,#9855,#9856);
#8573=AXIS2_PLACEMENT_3D('',#12324,#9858,#9859);
#8574=AXIS2_PLACEMENT_3D('',#12333,#9864,#9865);
#8575=AXIS2_PLACEMENT_3D('',#12339,#9869,#9870);
#8576=AXIS2_PLACEMENT_3D('',#12345,#9874,#9875);
#8577=AXIS2_PLACEMENT_3D('',#12348,#9878,#9879);
#8578=AXIS2_PLACEMENT_3D('',#12349,#9880,#9881);
#9719=DIRECTION('axis',(0.,0.,1.));
#9720=DIRECTION('refdir',(1.,0.,0.));
#9721=DIRECTION('center_axis',(0.,0.,1.));
#9722=DIRECTION('ref_axis',(1.,0.,0.));
#9723=DIRECTION('center_axis',(0.,0.,1.));
#9724=DIRECTION('ref_axis',(1.,0.,0.));
#9725=DIRECTION('',(0.,0.,1.));
#9726=DIRECTION('center_axis',(0.,0.,1.));
#9727=DIRECTION('ref_axis',(1.,0.,0.));
#9728=DIRECTION('center_axis',(0.,0.,1.));
#9729=DIRECTION('ref_axis',(1.,0.,0.));
#9730=DIRECTION('center_axis',(0.,0.,1.));
#9731=DIRECTION('ref_axis',(1.,0.,0.));
#9732=DIRECTION('center_axis',(0.,0.,1.));
#9733=DIRECTION('ref_axis',(1.,0.,0.));
#9734=DIRECTION('',(0.,0.,1.));
#9735=DIRECTION('center_axis',(0.,0.,1.));
#9736=DIRECTION('ref_axis',(1.,0.,0.));
#9737=DIRECTION('center_axis',(0.,0.,1.));
#9738=DIRECTION('ref_axis',(1.,0.,0.));
#9739=DIRECTION('center_axis',(0.,1.,0.));
#9740=DIRECTION('ref_axis',(1.,0.,0.));
#9741=DIRECTION('',(1.,0.,0.));
#9742=DIRECTION('center_axis',(0.,1.,0.));
#9743=DIRECTION('ref_axis',(1.,0.,0.));
#9744=DIRECTION('center_axis',(0.,1.,0.));
#9745=DIRECTION('ref_axis',(1.,0.,0.));
#9746=DIRECTION('',(0.,0.,1.));
#9747=DIRECTION('center_axis',(0.,1.,0.));
#9748=DIRECTION('ref_axis',(1.,0.,0.));
#9749=DIRECTION('center_axis',(0.,1.,0.));
#9750=DIRECTION('ref_axis',(1.,0.,0.));
#9751=DIRECTION('',(0.,0.,-1.));
#9752=DIRECTION('center_axis',(0.,1.,0.));
#9753=DIRECTION('ref_axis',(1.,0.,0.));
#9754=DIRECTION('center_axis',(0.,1.,0.));
#9755=DIRECTION('ref_axis',(1.,0.,0.));
#9756=DIRECTION('',(0.,1.,0.));
#9757=DIRECTION('center_axis',(0.,1.,0.));
#9758=DIRECTION('ref_axis',(1.,0.,0.));
#9759=DIRECTION('',(0.,-1.,0.));
#9760=DIRECTION('center_axis',(0.,1.,0.));
#9761=DIRECTION('ref_axis',(1.,0.,0.));
#9762=DIRECTION('',(0.,1.,0.));
#9763=DIRECTION('center_axis',(0.,-0.707106781186549,-0.707106781186546));
#9764=DIRECTION('ref_axis',(0.,0.707106781186546,-0.707106781186549));
#9765=DIRECTION('center_axis',(0.,-0.707106781186549,0.707106781186546));
#9766=DIRECTION('ref_axis',(0.,-0.707106781186546,-0.707106781186549));
#9767=DIRECTION('',(0.,-1.,0.));
#9768=DIRECTION('',(0.,1.,0.));
#9769=DIRECTION('center_axis',(0.,-0.707106781186549,0.707106781186546));
#9770=DIRECTION('ref_axis',(0.,-0.707106781186546,-0.707106781186549));
#9771=DIRECTION('center_axis',(0.,1.,0.));
#9772=DIRECTION('ref_axis',(1.,0.,0.));
#9773=DIRECTION('center_axis',(0.,1.,0.));
#9774=DIRECTION('ref_axis',(1.,0.,0.));
#9775=DIRECTION('center_axis',(0.,0.707106781186549,-0.707106781186546));
#9776=DIRECTION('ref_axis',(0.,-0.707106781186546,-0.707106781186549));
#9777=DIRECTION('center_axis',(0.,0.707106781186549,0.707106781186546));
#9778=DIRECTION('ref_axis',(0.,0.707106781186546,-0.707106781186549));
#9779=DIRECTION('center_axis',(0.,1.,0.));
#9780=DIRECTION('ref_axis',(-1.,0.,1.22464679914735E-16));
#9781=DIRECTION('center_axis',(0.,0.707106781186549,-0.707106781186546));
#9782=DIRECTION('ref_axis',(0.,-0.707106781186546,-0.707106781186549));
#9783=DIRECTION('center_axis',(0.,0.707106781186549,0.707106781186546));
#9784=DIRECTION('ref_axis',(0.,0.707106781186546,-0.707106781186549));
#9785=DIRECTION('center_axis',(0.,1.,0.));
#9786=DIRECTION('ref_axis',(1.,0.,0.));
#9787=DIRECTION('center_axis',(0.,1.,0.));
#9788=DIRECTION('ref_axis',(1.,0.,0.));
#9789=DIRECTION('center_axis',(0.,0.,1.));
#9790=DIRECTION('ref_axis',(1.,0.,0.));
#9791=DIRECTION('center_axis',(0.,0.,1.));
#9792=DIRECTION('ref_axis',(1.,0.,0.));
#9793=DIRECTION('center_axis',(0.,0.,1.));
#9794=DIRECTION('ref_axis',(1.,0.,0.));
#9795=DIRECTION('center_axis',(0.,0.,1.));
#9796=DIRECTION('ref_axis',(1.,0.,0.));
#9797=DIRECTION('center_axis',(0.,0.,1.));
#9798=DIRECTION('ref_axis',(1.,0.,0.));
#9799=DIRECTION('center_axis',(0.,0.,1.));
#9800=DIRECTION('ref_axis',(1.,0.,0.));
#9801=DIRECTION('center_axis',(0.,0.,1.));
#9802=DIRECTION('ref_axis',(1.,0.,0.));
#9803=DIRECTION('center_axis',(0.,0.,1.));
#9804=DIRECTION('ref_axis',(-1.,5.20660583828602E-15,0.));
#9805=DIRECTION('center_axis',(0.,0.,1.));
#9806=DIRECTION('ref_axis',(1.,0.,0.));
#9807=DIRECTION('',(0.,0.,1.));
#9808=DIRECTION('center_axis',(0.,0.,-1.));
#9809=DIRECTION('ref_axis',(1.,0.,0.));
#9810=DIRECTION('center_axis',(0.,1.,0.));
#9811=DIRECTION('ref_axis',(1.,0.,0.));
#9812=DIRECTION('center_axis',(0.,1.,0.));
#9813=DIRECTION('ref_axis',(1.,0.,0.));
#9814=DIRECTION('center_axis',(0.,1.,0.));
#9815=DIRECTION('ref_axis',(1.,0.,0.));
#9816=DIRECTION('center_axis',(0.,0.,1.));
#9817=DIRECTION('ref_axis',(1.,0.,0.));
#9818=DIRECTION('center_axis',(0.,0.,1.));
#9819=DIRECTION('ref_axis',(1.,0.,0.));
#9820=DIRECTION('',(0.,0.,1.));
#9821=DIRECTION('center_axis',(0.,0.,-1.));
#9822=DIRECTION('ref_axis',(1.,0.,0.));
#9823=DIRECTION('center_axis',(0.,0.,1.));
#9824=DIRECTION('ref_axis',(1.,0.,0.));
#9825=DIRECTION('center_axis',(0.,1.,0.));
#9826=DIRECTION('ref_axis',(1.,0.,0.));
#9827=DIRECTION('center_axis',(0.,1.,0.));
#9828=DIRECTION('ref_axis',(1.,0.,0.));
#9829=DIRECTION('',(0.,1.,0.));
#9830=DIRECTION('center_axis',(0.,-1.,0.));
#9831=DIRECTION('ref_axis',(1.,0.,0.));
#9832=DIRECTION('center_axis',(0.,1.,0.));
#9833=DIRECTION('ref_axis',(1.,0.,0.));
#9834=DIRECTION('center_axis',(0.,1.,0.));
#9835=DIRECTION('ref_axis',(1.,0.,0.));
#9836=DIRECTION('',(0.,1.,0.));
#9837=DIRECTION('center_axis',(0.,-1.,0.));
#9838=DIRECTION('ref_axis',(1.,0.,0.));
#9839=DIRECTION('center_axis',(0.,1.,0.));
#9840=DIRECTION('ref_axis',(1.,0.,0.));
#9841=DIRECTION('center_axis',(0.,1.,0.));
#9842=DIRECTION('ref_axis',(1.,0.,0.));
#9843=DIRECTION('',(0.,1.,0.));
#9844=DIRECTION('center_axis',(0.,-1.,0.));
#9845=DIRECTION('ref_axis',(1.,0.,0.));
#9846=DIRECTION('center_axis',(0.,1.,0.));
#9847=DIRECTION('ref_axis',(1.,0.,0.));
#9848=DIRECTION('center_axis',(0.,1.,0.));
#9849=DIRECTION('ref_axis',(1.,0.,0.));
#9850=DIRECTION('',(0.,1.,0.));
#9851=DIRECTION('center_axis',(0.,-1.,0.));
#9852=DIRECTION('ref_axis',(1.,0.,0.));
#9853=DIRECTION('center_axis',(0.,1.,0.));
#9854=DIRECTION('ref_axis',(1.,0.,0.));
#9855=DIRECTION('center_axis',(0.,1.,0.));
#9856=DIRECTION('ref_axis',(1.,0.,0.));
#9857=DIRECTION('',(0.,1.,0.));
#9858=DIRECTION('center_axis',(0.,1.,0.));
#9859=DIRECTION('ref_axis',(-1.,0.,0.));
#9860=DIRECTION('',(-1.,0.,0.));
#9861=DIRECTION('',(0.,0.,1.));
#9862=DIRECTION('',(-1.,0.,0.));
#9863=DIRECTION('',(0.,0.,1.));
#9864=DIRECTION('center_axis',(1.,0.,0.));
#9865=DIRECTION('ref_axis',(0.,1.,0.));
#9866=DIRECTION('',(0.,1.,0.));
#9867=DIRECTION('',(0.,1.,0.));
#9868=DIRECTION('',(0.,0.,1.));
#9869=DIRECTION('center_axis',(0.,-1.,0.));
#9870=DIRECTION('ref_axis',(1.,0.,0.));
#9871=DIRECTION('',(1.,0.,0.));
#9872=DIRECTION('',(1.,0.,0.));
#9873=DIRECTION('',(0.,0.,1.));
#9874=DIRECTION('center_axis',(-1.,0.,0.));
#9875=DIRECTION('ref_axis',(0.,-1.,0.));
#9876=DIRECTION('',(0.,-1.,0.));
#9877=DIRECTION('',(0.,-1.,0.));
#9878=DIRECTION('center_axis',(0.,0.,1.));
#9879=DIRECTION('ref_axis',(1.,0.,0.));
#9880=DIRECTION('center_axis',(0.,0.,1.));
#9881=DIRECTION('ref_axis',(1.,0.,0.));
#12216=CARTESIAN_POINT('',(0.,0.,0.));
#12217=CARTESIAN_POINT('Origin',(-1.2,12.,1.9));
#12218=CARTESIAN_POINT('',(-1.41,12.,2.));
#12219=CARTESIAN_POINT('Origin',(-1.2,12.,2.));
#12220=CARTESIAN_POINT('',(-1.41,12.,3.1));
#12221=CARTESIAN_POINT('',(-1.41,12.,1.9));
#12222=CARTESIAN_POINT('Origin',(-1.2,12.,3.1));
#12223=CARTESIAN_POINT('Origin',(-1.2,12.,3.1));
#12224=CARTESIAN_POINT('Origin',(1.2,12.,1.9));
#12225=CARTESIAN_POINT('',(0.99,12.,2.));
#12226=CARTESIAN_POINT('Origin',(1.2,12.,2.));
#12227=CARTESIAN_POINT('',(0.99,12.,3.1));
#12228=CARTESIAN_POINT('',(0.99,12.,1.9));
#12229=CARTESIAN_POINT('Origin',(1.2,12.,3.1));
#12230=CARTESIAN_POINT('Origin',(1.2,12.,3.1));
#12231=CARTESIAN_POINT('Origin',(0.,11.9,5.4));
#12232=CARTESIAN_POINT('',(-0.173205080756887,11.9,5.3));
#12233=CARTESIAN_POINT('',(0.173205080756887,11.9,5.3));
#12234=CARTESIAN_POINT('',(0.,11.9,5.3));
#12235=CARTESIAN_POINT('Origin',(0.,11.9,5.4));
#12236=CARTESIAN_POINT('Origin',(0.,11.9,5.4));
#12237=CARTESIAN_POINT('',(0.173205080756887,11.9,5.5));
#12238=CARTESIAN_POINT('',(0.173205080756887,11.9,5.3));
#12239=CARTESIAN_POINT('Origin',(0.,11.9,5.4));
#12240=CARTESIAN_POINT('Origin',(0.,11.9,5.4));
#12241=CARTESIAN_POINT('',(-0.173205080756887,11.9,5.5));
#12242=CARTESIAN_POINT('',(-0.173205080756887,11.9,5.3));
#12243=CARTESIAN_POINT('Origin',(0.,11.9,5.4));
#12244=CARTESIAN_POINT('Origin',(0.,11.1,5.4));
#12245=CARTESIAN_POINT('',(0.181811868577262,11.1,5.48333333333333));
#12246=CARTESIAN_POINT('',(0.181811868577262,11.4,5.48333333333333));
#12247=CARTESIAN_POINT('',(0.181811868577262,11.1,5.48333333333333));
#12248=CARTESIAN_POINT('',(-0.181811868577262,11.1,5.48333333333333));
#12249=CARTESIAN_POINT('Origin',(0.,11.1,5.4));
#12250=CARTESIAN_POINT('',(-0.181811868577262,11.4,5.48333333333333));
#12251=CARTESIAN_POINT('',(-0.181811868577262,11.1,5.48333333333333));
#12252=CARTESIAN_POINT('',(-0.2,11.4,5.4));
#12253=CARTESIAN_POINT('Origin',(0.,11.4,5.4));
#12254=CARTESIAN_POINT('',(-0.2,11.8,5.4));
#12255=CARTESIAN_POINT('',(-0.2,11.1,5.4));
#12256=CARTESIAN_POINT('',(0.2,11.8,5.4));
#12257=CARTESIAN_POINT('Origin',(0.,11.8,5.4));
#12258=CARTESIAN_POINT('',(0.173205080756888,11.7,5.3));
#12259=CARTESIAN_POINT('Origin',(0.,11.8,5.4));
#12260=CARTESIAN_POINT('',(0.173205080756888,11.1,5.3));
#12261=CARTESIAN_POINT('',(-0.173205080756888,11.7,5.3));
#12262=CARTESIAN_POINT('',(-0.173205080756888,11.1,5.3));
#12263=CARTESIAN_POINT('Origin',(0.,11.8,5.4));
#12264=CARTESIAN_POINT('Origin',(0.,11.4,5.4));
#12265=CARTESIAN_POINT('Origin',(0.,11.1,5.4));
#12266=CARTESIAN_POINT('Origin',(0.,11.8,5.4));
#12267=CARTESIAN_POINT('Origin',(0.,11.8,5.4));
#12268=CARTESIAN_POINT('Origin',(0.,11.1,5.4));
#12269=CARTESIAN_POINT('Origin',(0.,11.8,5.4));
#12270=CARTESIAN_POINT('Origin',(0.,11.8,5.4));
#12271=CARTESIAN_POINT('Origin',(0.,11.1,5.4));
#12272=CARTESIAN_POINT('Origin',(0.,11.1,4.5));
#12273=CARTESIAN_POINT('Origin',(0.,11.8,5.3));
#12274=CARTESIAN_POINT('Origin',(0.,11.8,5.3));
#12275=CARTESIAN_POINT('Origin',(0.,11.8,5.3));
#12276=CARTESIAN_POINT('Origin',(0.,11.8,5.3));
#12277=CARTESIAN_POINT('Origin',(0.,11.8,5.3));
#12278=CARTESIAN_POINT('Origin',(0.,11.8,5.3));
#12279=CARTESIAN_POINT('Origin',(0.,11.8,5.3));
#12280=CARTESIAN_POINT('Origin',(0.,11.8,5.3));
#12281=CARTESIAN_POINT('Origin',(0.,11.8,5.3));
#12282=CARTESIAN_POINT('',(-0.2,11.8,5.8));
#12283=CARTESIAN_POINT('',(-0.2,11.8,5.3));
#12284=CARTESIAN_POINT('Origin',(0.,11.8,5.8));
#12285=CARTESIAN_POINT('Origin',(0.,11.4,4.5));
#12286=CARTESIAN_POINT('',(-1.,11.4,4.5));
#12287=CARTESIAN_POINT('Origin',(0.,11.4,4.5));
#12288=CARTESIAN_POINT('Origin',(0.,11.4,4.5));
#12289=CARTESIAN_POINT('Origin',(0.,11.8,5.8));
#12290=CARTESIAN_POINT('',(-0.685,11.8,5.8));
#12291=CARTESIAN_POINT('Origin',(0.,11.8,5.8));
#12292=CARTESIAN_POINT('',(-0.685,11.8,7.));
#12293=CARTESIAN_POINT('',(-0.685,11.8,5.8));
#12294=CARTESIAN_POINT('Origin',(0.,11.8,7.));
#12295=CARTESIAN_POINT('Origin',(0.,11.8,5.8));
#12296=CARTESIAN_POINT('Origin',(2.,10.8,2.5));
#12297=CARTESIAN_POINT('',(1.725,10.9,2.5));
#12298=CARTESIAN_POINT('Origin',(2.,10.9,2.5));
#12299=CARTESIAN_POINT('',(1.725,12.6,2.5));
#12300=CARTESIAN_POINT('',(1.725,10.8,2.5));
#12301=CARTESIAN_POINT('Origin',(2.,12.6,2.5));
#12302=CARTESIAN_POINT('Origin',(-2.,10.8,6.5));
#12303=CARTESIAN_POINT('',(-2.275,10.9,6.5));
#12304=CARTESIAN_POINT('Origin',(-2.,10.9,6.5));
#12305=CARTESIAN_POINT('',(-2.275,12.6,6.5));
#12306=CARTESIAN_POINT('',(-2.275,10.8,6.5));
#12307=CARTESIAN_POINT('Origin',(-2.,12.6,6.5));
#12308=CARTESIAN_POINT('Origin',(-2.,10.8,2.5));
#12309=CARTESIAN_POINT('',(-2.275,10.9,2.5));
#12310=CARTESIAN_POINT('Origin',(-2.,10.9,2.5));
#12311=CARTESIAN_POINT('',(-2.275,12.6,2.5));
#12312=CARTESIAN_POINT('',(-2.275,10.8,2.5));
#12313=CARTESIAN_POINT('Origin',(-2.,12.6,2.5));
#12314=CARTESIAN_POINT('Origin',(2.,10.8,6.5));
#12315=CARTESIAN_POINT('',(1.725,10.9,6.5));
#12316=CARTESIAN_POINT('Origin',(2.,10.9,6.5));
#12317=CARTESIAN_POINT('',(1.725,12.6,6.5));
#12318=CARTESIAN_POINT('',(1.725,10.8,6.5));
#12319=CARTESIAN_POINT('Origin',(2.,12.6,6.5));
#12320=CARTESIAN_POINT('Origin',(0.,10.8,4.5));
#12321=CARTESIAN_POINT('',(-1.,10.9,4.5));
#12322=CARTESIAN_POINT('Origin',(0.,10.9,4.5));
#12323=CARTESIAN_POINT('',(-1.,10.8,4.5));
#12324=CARTESIAN_POINT('Origin',(2.5,12.6,2.));
#12325=CARTESIAN_POINT('',(2.5,12.6,2.));
#12326=CARTESIAN_POINT('',(-2.5,12.6,2.));
#12327=CARTESIAN_POINT('',(2.5,12.6,2.));
#12328=CARTESIAN_POINT('',(-2.5,12.6,7.));
#12329=CARTESIAN_POINT('',(-2.5,12.6,2.));
#12330=CARTESIAN_POINT('',(2.5,12.6,7.));
#12331=CARTESIAN_POINT('',(2.5,12.6,7.));
#12332=CARTESIAN_POINT('',(2.5,12.6,2.));
#12333=CARTESIAN_POINT('Origin',(2.5,10.9,2.));
#12334=CARTESIAN_POINT('',(2.5,10.9,2.));
#12335=CARTESIAN_POINT('',(2.5,10.9,2.));
#12336=CARTESIAN_POINT('',(2.5,10.9,7.));
#12337=CARTESIAN_POINT('',(2.5,10.9,7.));
#12338=CARTESIAN_POINT('',(2.5,10.9,2.));
#12339=CARTESIAN_POINT('Origin',(-2.5,10.9,2.));
#12340=CARTESIAN_POINT('',(-2.5,10.9,2.));
#12341=CARTESIAN_POINT('',(-2.5,10.9,2.));
#12342=CARTESIAN_POINT('',(-2.5,10.9,7.));
#12343=CARTESIAN_POINT('',(-2.5,10.9,7.));
#12344=CARTESIAN_POINT('',(-2.5,10.9,2.));
#12345=CARTESIAN_POINT('Origin',(-2.5,12.6,2.));
#12346=CARTESIAN_POINT('',(-2.5,12.6,2.));
#12347=CARTESIAN_POINT('',(-2.5,12.6,7.));
#12348=CARTESIAN_POINT('Origin',(0.,11.75,7.));
#12349=CARTESIAN_POINT('Origin',(0.,11.75,2.));
#14302=UNCERTAINTY_MEASURE_WITH_UNIT(LENGTH_MEASURE(0.001),#14393,
'DISTANCE_ACCURACY_VALUE',
'Maximum model space distance between geometric entities at asserted c
onnectivities');
#14344=UNCERTAINTY_MEASURE_WITH_UNIT(LENGTH_MEASURE(0.001),#14393,
'DISTANCE_ACCURACY_VALUE',
'Maximum model space distance between geometric entities at asserted c
onnectivities');
#14350=(
GEOMETRIC_REPRESENTATION_CONTEXT(3)
GLOBAL_UNCERTAINTY_ASSIGNED_CONTEXT((#14302))
GLOBAL_UNIT_ASSIGNED_CONTEXT((#14393,#14395,#14396))
REPRESENTATION_CONTEXT('','3D')
);
#14392=(
GEOMETRIC_REPRESENTATION_CONTEXT(3)
GLOBAL_UNCERTAINTY_ASSIGNED_CONTEXT((#14344))
GLOBAL_UNIT_ASSIGNED_CONTEXT((#14393,#14395,#14396))
REPRESENTATION_CONTEXT('','3D')
);
#14393=(
LENGTH_UNIT()
NAMED_UNIT(*)
SI_UNIT(.CENTI.,.METRE.)
);
#14395=(
NAMED_UNIT(*)
PLANE_ANGLE_UNIT()
SI_UNIT($,.RADIAN.)
);
#14396=(
NAMED_UNIT(*)
SI_UNIT($,.STERADIAN.)
SOLID_ANGLE_UNIT()
);
#14402=SHAPE_DEFINITION_REPRESENTATION(#14449,#14588);
#14449=PRODUCT_DEFINITION_SHAPE('',$,#14636);
#14588=SHAPE_REPRESENTATION('',(#8512),#14350);
#14630=PRODUCT_DEFINITION_CONTEXT('part definition',#14773,'design');
#14636=PRODUCT_DEFINITION('Rear cylinder cap','Rear cylinder cap',#14683,
#14630);
#14683=PRODUCT_DEFINITION_FORMATION('',$,#14780);
#14773=APPLICATION_CONTEXT(
'Core Data for Automotive Mechanical Design Process');
#14774=PRODUCT_CONTEXT('part definition',#14773,'mechanical');
#14780=PRODUCT('Rear cylinder cap','Rear cylinder cap',
'Rear cylinder cap',(#14774));
#14871=COLOUR_RGB('Light Blue',0.38,0.62,0.78);
#14872=FILL_AREA_STYLE_COLOUR('',#14871);
#14873=FILL_AREA_STYLE('',(#14872));
#14874=SURFACE_STYLE_FILL_AREA(#14873);
#14875=SURFACE_SIDE_STYLE('',(#14874));
#14876=SURFACE_STYLE_USAGE(.BOTH.,#14875);
#14877=PRESENTATION_STYLE_ASSIGNMENT((#14876));
ENDSEC;
END-ISO-10303-21;
